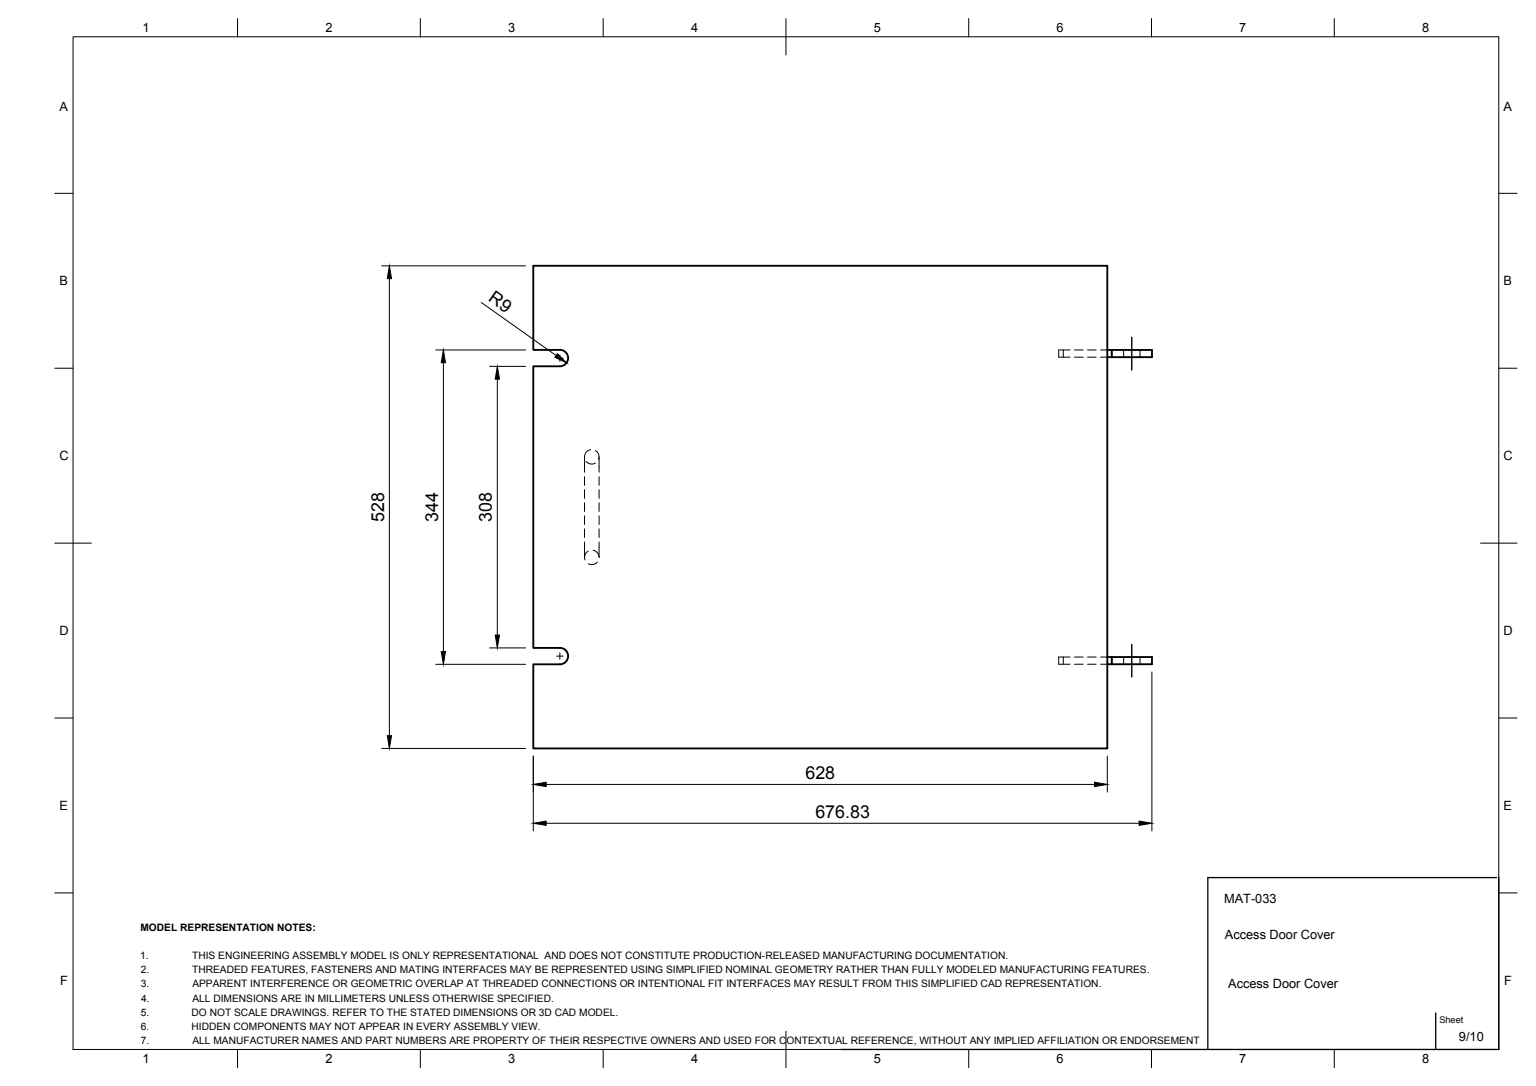
ISO-10303-21;
HEADER;
/* Generated by software containing ST-Developer
 * from STEP Tools, Inc. (www.steptools.com) 
 */

FILE_DESCRIPTION(
/* description */ ('STEP AP214'),
/* implementation_level */ '2;1');

FILE_NAME(
/* name */ 'Access Door Cover.step',
/* time_stamp */ '2026-11-14T07:13:32-08:00',
/* author */ (''),
/* organization */ (''),
/* preprocessor_version */ 'ST-DEVELOPER v20.2',
/* originating_system */ 'Autodesk Translation Framework v15.17.0.0',
/* authorisation */ '');

FILE_SCHEMA (('AUTOMOTIVE_DESIGN { 1 0 10303 214 3 1 1 }'));
ENDSEC;

DATA;
#10=MECHANICAL_DESIGN_GEOMETRIC_PRESENTATION_REPRESENTATION('',(#1315,#1316,#1317,#1318),#32903);
#639=TOROIDAL_SURFACE('',#16259,11.,7.93749999999998);
#640=TOROIDAL_SURFACE('',#16264,11.,7.93749999999998);
#675=SHAPE_REPRESENTATION_RELATIONSHIP('SRR','None',#33017,#689);
#689=ADVANCED_BREP_SHAPE_REPRESENTATION('',(#1404,#1405,#1406,#1407),#32892);
#856=CIRCLE('',#16214,9.00000000000001);
#857=CIRCLE('',#16215,9.00000000000001);
#858=CIRCLE('',#16220,9.00000000000001);
#859=CIRCLE('',#16221,9.00000000000001);
#860=CIRCLE('',#16230,9.00000000000001);
#861=CIRCLE('',#16231,9.00000000000001);
#862=CIRCLE('',#16233,5.);
#863=CIRCLE('',#16234,5.);
#864=CIRCLE('',#16236,22.);
#865=CIRCLE('',#16237,22.);
#866=CIRCLE('',#16245,9.00000000000001);
#867=CIRCLE('',#16246,9.00000000000001);
#868=CIRCLE('',#16248,5.);
#869=CIRCLE('',#16249,5.);
#870=CIRCLE('',#16251,22.);
#871=CIRCLE('',#16252,22.);
#872=CIRCLE('',#16260,7.93749999999998);
#873=CIRCLE('',#16261,3.06250000000001);
#874=CIRCLE('',#16262,7.93749999999998);
#875=CIRCLE('',#16263,7.93749999999998);
#876=CIRCLE('',#16265,7.93749999999998);
#877=CIRCLE('',#16266,3.06250000000001);
#878=CIRCLE('',#16267,7.93749999999998);
#879=CIRCLE('',#16268,7.93749999999998);
#880=CIRCLE('',#16270,7.93749999999998);
#881=CIRCLE('',#16273,7.93749999999998);
#1171=CYLINDRICAL_SURFACE('',#16213,9.00000000000001);
#1172=CYLINDRICAL_SURFACE('',#16219,9.00000000000001);
#1173=CYLINDRICAL_SURFACE('',#16229,9.00000000000001);
#1174=CYLINDRICAL_SURFACE('',#16232,5.);
#1175=CYLINDRICAL_SURFACE('',#16235,22.);
#1176=CYLINDRICAL_SURFACE('',#16244,9.00000000000001);
#1177=CYLINDRICAL_SURFACE('',#16247,5.);
#1178=CYLINDRICAL_SURFACE('',#16250,22.);
#1179=CYLINDRICAL_SURFACE('',#16269,7.93749999999998);
#1180=CYLINDRICAL_SURFACE('',#16271,7.93749999999999);
#1181=CYLINDRICAL_SURFACE('',#16272,7.93749999999998);
#1315=STYLED_ITEM('',(#33098),#1404);
#1316=STYLED_ITEM('',(#33098),#1405);
#1317=STYLED_ITEM('',(#33098),#1406);
#1318=STYLED_ITEM('',(#33098),#1407);
#1404=MANIFOLD_SOLID_BREP('Body1',#15563);
#1405=MANIFOLD_SOLID_BREP('Body2',#15564);
#1406=MANIFOLD_SOLID_BREP('Body3',#15565);
#1407=MANIFOLD_SOLID_BREP('Body4',#15566);
#1591=FACE_BOUND('',#2953,.T.);
#1592=FACE_BOUND('',#2955,.T.);
#1593=FACE_BOUND('',#2964,.T.);
#1594=FACE_BOUND('',#2966,.T.);
#1918=FACE_OUTER_BOUND('',#2935,.T.);
#1919=FACE_OUTER_BOUND('',#2936,.T.);
#1920=FACE_OUTER_BOUND('',#2937,.T.);
#1921=FACE_OUTER_BOUND('',#2938,.T.);
#1922=FACE_OUTER_BOUND('',#2939,.T.);
#1923=FACE_OUTER_BOUND('',#2940,.T.);
#1924=FACE_OUTER_BOUND('',#2941,.T.);
#1925=FACE_OUTER_BOUND('',#2942,.T.);
#1926=FACE_OUTER_BOUND('',#2943,.T.);
#1927=FACE_OUTER_BOUND('',#2944,.T.);
#1928=FACE_OUTER_BOUND('',#2945,.T.);
#1929=FACE_OUTER_BOUND('',#2946,.T.);
#1930=FACE_OUTER_BOUND('',#2947,.T.);
#1931=FACE_OUTER_BOUND('',#2948,.T.);
#1932=FACE_OUTER_BOUND('',#2949,.T.);
#1933=FACE_OUTER_BOUND('',#2950,.T.);
#1934=FACE_OUTER_BOUND('',#2951,.T.);
#1935=FACE_OUTER_BOUND('',#2952,.T.);
#1936=FACE_OUTER_BOUND('',#2954,.T.);
#1937=FACE_OUTER_BOUND('',#2956,.T.);
#1938=FACE_OUTER_BOUND('',#2957,.T.);
#1939=FACE_OUTER_BOUND('',#2958,.T.);
#1940=FACE_OUTER_BOUND('',#2959,.T.);
#1941=FACE_OUTER_BOUND('',#2960,.T.);
#1942=FACE_OUTER_BOUND('',#2961,.T.);
#1943=FACE_OUTER_BOUND('',#2962,.T.);
#1944=FACE_OUTER_BOUND('',#2963,.T.);
#1945=FACE_OUTER_BOUND('',#2965,.T.);
#1946=FACE_OUTER_BOUND('',#2967,.T.);
#1947=FACE_OUTER_BOUND('',#2968,.T.);
#1948=FACE_OUTER_BOUND('',#2969,.T.);
#1949=FACE_OUTER_BOUND('',#2970,.T.);
#1950=FACE_OUTER_BOUND('',#2971,.T.);
#1951=FACE_OUTER_BOUND('',#2972,.T.);
#1952=FACE_OUTER_BOUND('',#2973,.T.);
#1953=FACE_OUTER_BOUND('',#2974,.T.);
#1954=FACE_OUTER_BOUND('',#2975,.T.);
#1955=FACE_OUTER_BOUND('',#2976,.T.);
#1956=FACE_OUTER_BOUND('',#2977,.T.);
#2935=EDGE_LOOP('',(#11071,#11072,#11073,#11074));
#2936=EDGE_LOOP('',(#11075,#11076,#11077,#11078));
#2937=EDGE_LOOP('',(#11079,#11080,#11081,#11082));
#2938=EDGE_LOOP('',(#11083,#11084,#11085,#11086));
#2939=EDGE_LOOP('',(#11087,#11088,#11089,#11090));
#2940=EDGE_LOOP('',(#11091,#11092,#11093,#11094));
#2941=EDGE_LOOP('',(#11095,#11096,#11097,#11098));
#2942=EDGE_LOOP('',(#11099,#11100,#11101,#11102));
#2943=EDGE_LOOP('',(#11103,#11104,#11105,#11106));
#2944=EDGE_LOOP('',(#11107,#11108,#11109,#11110));
#2945=EDGE_LOOP('',(#11111,#11112,#11113,#11114));
#2946=EDGE_LOOP('',(#11115,#11116,#11117,#11118));
#2947=EDGE_LOOP('',(#11119,#11120,#11121,#11122,#11123,#11124,#11125,#11126,
#11127,#11128,#11129,#11130));
#2948=EDGE_LOOP('',(#11131,#11132,#11133,#11134,#11135,#11136,#11137,#11138,
#11139,#11140,#11141,#11142));
#2949=EDGE_LOOP('',(#11143,#11144,#11145,#11146));
#2950=EDGE_LOOP('',(#11147,#11148,#11149,#11150));
#2951=EDGE_LOOP('',(#11151,#11152,#11153,#11154));
#2952=EDGE_LOOP('',(#11155,#11156,#11157,#11158,#11159,#11160));
#2953=EDGE_LOOP('',(#11161));
#2954=EDGE_LOOP('',(#11162,#11163,#11164,#11165,#11166,#11167));
#2955=EDGE_LOOP('',(#11168));
#2956=EDGE_LOOP('',(#11169,#11170,#11171,#11172));
#2957=EDGE_LOOP('',(#11173,#11174,#11175,#11176));
#2958=EDGE_LOOP('',(#11177,#11178,#11179,#11180));
#2959=EDGE_LOOP('',(#11181,#11182,#11183,#11184));
#2960=EDGE_LOOP('',(#11185,#11186,#11187,#11188));
#2961=EDGE_LOOP('',(#11189,#11190,#11191,#11192));
#2962=EDGE_LOOP('',(#11193,#11194,#11195,#11196));
#2963=EDGE_LOOP('',(#11197,#11198,#11199,#11200,#11201,#11202));
#2964=EDGE_LOOP('',(#11203));
#2965=EDGE_LOOP('',(#11204,#11205,#11206,#11207,#11208,#11209));
#2966=EDGE_LOOP('',(#11210));
#2967=EDGE_LOOP('',(#11211,#11212,#11213,#11214));
#2968=EDGE_LOOP('',(#11215,#11216,#11217,#11218));
#2969=EDGE_LOOP('',(#11219,#11220,#11221,#11222));
#2970=EDGE_LOOP('',(#11223,#11224,#11225,#11226));
#2971=EDGE_LOOP('',(#11227,#11228,#11229,#11230,#11231));
#2972=EDGE_LOOP('',(#11232,#11233,#11234,#11235,#11236));
#2973=EDGE_LOOP('',(#11237,#11238,#11239,#11240));
#2974=EDGE_LOOP('',(#11241,#11242,#11243,#11244,#11245,#11246));
#2975=EDGE_LOOP('',(#11247,#11248,#11249,#11250));
#2976=EDGE_LOOP('',(#11251));
#2977=EDGE_LOOP('',(#11252));
#4075=LINE('',#22530,#5479);
#4076=LINE('',#22532,#5480);
#4077=LINE('',#22534,#5481);
#4078=LINE('',#22535,#5482);
#4079=LINE('',#22538,#5483);
#4080=LINE('',#22540,#5484);
#4081=LINE('',#22541,#5485);
#4082=LINE('',#22546,#5486);
#4083=LINE('',#22550,#5487);
#4084=LINE('',#22552,#5488);
#4085=LINE('',#22553,#5489);
#4086=LINE('',#22556,#5490);
#4087=LINE('',#22558,#5491);
#4088=LINE('',#22559,#5492);
#4089=LINE('',#22562,#5493);
#4090=LINE('',#22564,#5494);
#4091=LINE('',#22565,#5495);
#4092=LINE('',#22570,#5496);
#4093=LINE('',#22574,#5497);
#4094=LINE('',#22576,#5498);
#4095=LINE('',#22577,#5499);
#4096=LINE('',#22580,#5500);
#4097=LINE('',#22582,#5501);
#4098=LINE('',#22583,#5502);
#4099=LINE('',#22586,#5503);
#4100=LINE('',#22588,#5504);
#4101=LINE('',#22589,#5505);
#4102=LINE('',#22592,#5506);
#4103=LINE('',#22594,#5507);
#4104=LINE('',#22595,#5508);
#4105=LINE('',#22597,#5509);
#4106=LINE('',#22598,#5510);
#4107=LINE('',#22605,#5511);
#4108=LINE('',#22612,#5512);
#4109=LINE('',#22615,#5513);
#4110=LINE('',#22620,#5514);
#4111=LINE('',#22624,#5515);
#4112=LINE('',#22626,#5516);
#4113=LINE('',#22628,#5517);
#4114=LINE('',#22629,#5518);
#4115=LINE('',#22632,#5519);
#4116=LINE('',#22634,#5520);
#4117=LINE('',#22636,#5521);
#4118=LINE('',#22637,#5522);
#4119=LINE('',#22639,#5523);
#4120=LINE('',#22641,#5524);
#4121=LINE('',#22643,#5525);
#4122=LINE('',#22649,#5526);
#4123=LINE('',#22656,#5527);
#4124=LINE('',#22659,#5528);
#4125=LINE('',#22665,#5529);
#4126=LINE('',#22668,#5530);
#4127=LINE('',#22670,#5531);
#4128=LINE('',#22672,#5532);
#4129=LINE('',#22673,#5533);
#4130=LINE('',#22676,#5534);
#4131=LINE('',#22678,#5535);
#4132=LINE('',#22680,#5536);
#4133=LINE('',#22681,#5537);
#4134=LINE('',#22683,#5538);
#4135=LINE('',#22685,#5539);
#4136=LINE('',#22687,#5540);
#4137=LINE('',#22707,#5541);
#4138=LINE('',#22710,#5542);
#4139=LINE('',#22714,#5543);
#5479=VECTOR('',#18417,1000.);
#5480=VECTOR('',#18418,1000.);
#5481=VECTOR('',#18419,1000.);
#5482=VECTOR('',#18420,1000.);
#5483=VECTOR('',#18423,1000.);
#5484=VECTOR('',#18424,1000.);
#5485=VECTOR('',#18425,1000.);
#5486=VECTOR('',#18430,1000.);
#5487=VECTOR('',#18435,1000.);
#5488=VECTOR('',#18436,1000.);
#5489=VECTOR('',#18437,1000.);
#5490=VECTOR('',#18440,1000.);
#5491=VECTOR('',#18441,1000.);
#5492=VECTOR('',#18442,1000.);
#5493=VECTOR('',#18445,1000.);
#5494=VECTOR('',#18446,1000.);
#5495=VECTOR('',#18447,1000.);
#5496=VECTOR('',#18452,1000.);
#5497=VECTOR('',#18457,1000.);
#5498=VECTOR('',#18458,1000.);
#5499=VECTOR('',#18459,1000.);
#5500=VECTOR('',#18462,1000.);
#5501=VECTOR('',#18463,1000.);
#5502=VECTOR('',#18464,1000.);
#5503=VECTOR('',#18467,1000.);
#5504=VECTOR('',#18468,1000.);
#5505=VECTOR('',#18469,1000.);
#5506=VECTOR('',#18472,1000.);
#5507=VECTOR('',#18473,1000.);
#5508=VECTOR('',#18474,1000.);
#5509=VECTOR('',#18477,1000.);
#5510=VECTOR('',#18478,1000.);
#5511=VECTOR('',#18487,9.00000000000001);
#5512=VECTOR('',#18494,1000.);
#5513=VECTOR('',#18497,1000.);
#5514=VECTOR('',#18502,1000.);
#5515=VECTOR('',#18507,1000.);
#5516=VECTOR('',#18508,1000.);
#5517=VECTOR('',#18509,1000.);
#5518=VECTOR('',#18510,1000.);
#5519=VECTOR('',#18513,1000.);
#5520=VECTOR('',#18514,1000.);
#5521=VECTOR('',#18515,1000.);
#5522=VECTOR('',#18516,1000.);
#5523=VECTOR('',#18519,1000.);
#5524=VECTOR('',#18522,1000.);
#5525=VECTOR('',#18525,1000.);
#5526=VECTOR('',#18532,9.00000000000001);
#5527=VECTOR('',#18539,1000.);
#5528=VECTOR('',#18542,1000.);
#5529=VECTOR('',#18549,1000.);
#5530=VECTOR('',#18552,1000.);
#5531=VECTOR('',#18553,1000.);
#5532=VECTOR('',#18554,1000.);
#5533=VECTOR('',#18555,1000.);
#5534=VECTOR('',#18558,1000.);
#5535=VECTOR('',#18559,1000.);
#5536=VECTOR('',#18560,1000.);
#5537=VECTOR('',#18561,1000.);
#5538=VECTOR('',#18564,1000.);
#5539=VECTOR('',#18567,1000.);
#5540=VECTOR('',#18570,1000.);
#5541=VECTOR('',#18595,7.93749999999998);
#5542=VECTOR('',#18600,7.93749999999999);
#5543=VECTOR('',#18605,7.93749999999998);
#6869=VERTEX_POINT('',#22528);
#6870=VERTEX_POINT('',#22529);
#6871=VERTEX_POINT('',#22531);
#6872=VERTEX_POINT('',#22533);
#6873=VERTEX_POINT('',#22537);
#6874=VERTEX_POINT('',#22539);
#6875=VERTEX_POINT('',#22543);
#6876=VERTEX_POINT('',#22545);
#6877=VERTEX_POINT('',#22549);
#6878=VERTEX_POINT('',#22551);
#6879=VERTEX_POINT('',#22555);
#6880=VERTEX_POINT('',#22557);
#6881=VERTEX_POINT('',#22561);
#6882=VERTEX_POINT('',#22563);
#6883=VERTEX_POINT('',#22567);
#6884=VERTEX_POINT('',#22569);
#6885=VERTEX_POINT('',#22573);
#6886=VERTEX_POINT('',#22575);
#6887=VERTEX_POINT('',#22579);
#6888=VERTEX_POINT('',#22581);
#6889=VERTEX_POINT('',#22585);
#6890=VERTEX_POINT('',#22587);
#6891=VERTEX_POINT('',#22591);
#6892=VERTEX_POINT('',#22593);
#6893=VERTEX_POINT('',#22602);
#6894=VERTEX_POINT('',#22604);
#6895=VERTEX_POINT('',#22608);
#6896=VERTEX_POINT('',#22609);
#6897=VERTEX_POINT('',#22611);
#6898=VERTEX_POINT('',#22613);
#6899=VERTEX_POINT('',#22617);
#6900=VERTEX_POINT('',#22619);
#6901=VERTEX_POINT('',#22623);
#6902=VERTEX_POINT('',#22625);
#6903=VERTEX_POINT('',#22627);
#6904=VERTEX_POINT('',#22631);
#6905=VERTEX_POINT('',#22633);
#6906=VERTEX_POINT('',#22635);
#6907=VERTEX_POINT('',#22646);
#6908=VERTEX_POINT('',#22648);
#6909=VERTEX_POINT('',#22652);
#6910=VERTEX_POINT('',#22653);
#6911=VERTEX_POINT('',#22655);
#6912=VERTEX_POINT('',#22657);
#6913=VERTEX_POINT('',#22661);
#6914=VERTEX_POINT('',#22663);
#6915=VERTEX_POINT('',#22667);
#6916=VERTEX_POINT('',#22669);
#6917=VERTEX_POINT('',#22671);
#6918=VERTEX_POINT('',#22675);
#6919=VERTEX_POINT('',#22677);
#6920=VERTEX_POINT('',#22679);
#6921=VERTEX_POINT('',#22690);
#6922=VERTEX_POINT('',#22691);
#6923=VERTEX_POINT('',#22693);
#6924=VERTEX_POINT('',#22698);
#6925=VERTEX_POINT('',#22700);
#6926=VERTEX_POINT('',#22702);
#6927=VERTEX_POINT('',#22706);
#6928=VERTEX_POINT('',#22712);
#8419=EDGE_CURVE('',#6869,#6870,#4075,.T.);
#8420=EDGE_CURVE('',#6871,#6869,#4076,.T.);
#8421=EDGE_CURVE('',#6871,#6872,#4077,.T.);
#8422=EDGE_CURVE('',#6872,#6870,#4078,.T.);
#8423=EDGE_CURVE('',#6873,#6869,#4079,.T.);
#8424=EDGE_CURVE('',#6874,#6873,#4080,.T.);
#8425=EDGE_CURVE('',#6874,#6871,#4081,.T.);
#8426=EDGE_CURVE('',#6875,#6873,#856,.T.);
#8427=EDGE_CURVE('',#6876,#6875,#4082,.T.);
#8428=EDGE_CURVE('',#6876,#6874,#857,.T.);
#8429=EDGE_CURVE('',#6877,#6875,#4083,.T.);
#8430=EDGE_CURVE('',#6878,#6877,#4084,.T.);
#8431=EDGE_CURVE('',#6878,#6876,#4085,.T.);
#8432=EDGE_CURVE('',#6879,#6877,#4086,.T.);
#8433=EDGE_CURVE('',#6880,#6879,#4087,.T.);
#8434=EDGE_CURVE('',#6880,#6878,#4088,.T.);
#8435=EDGE_CURVE('',#6881,#6879,#4089,.T.);
#8436=EDGE_CURVE('',#6882,#6881,#4090,.T.);
#8437=EDGE_CURVE('',#6882,#6880,#4091,.T.);
#8438=EDGE_CURVE('',#6883,#6881,#858,.T.);
#8439=EDGE_CURVE('',#6884,#6883,#4092,.T.);
#8440=EDGE_CURVE('',#6884,#6882,#859,.T.);
#8441=EDGE_CURVE('',#6885,#6883,#4093,.T.);
#8442=EDGE_CURVE('',#6886,#6885,#4094,.T.);
#8443=EDGE_CURVE('',#6886,#6884,#4095,.T.);
#8444=EDGE_CURVE('',#6887,#6885,#4096,.T.);
#8445=EDGE_CURVE('',#6888,#6887,#4097,.T.);
#8446=EDGE_CURVE('',#6888,#6886,#4098,.T.);
#8447=EDGE_CURVE('',#6889,#6887,#4099,.T.);
#8448=EDGE_CURVE('',#6890,#6889,#4100,.T.);
#8449=EDGE_CURVE('',#6890,#6888,#4101,.T.);
#8450=EDGE_CURVE('',#6891,#6889,#4102,.T.);
#8451=EDGE_CURVE('',#6892,#6891,#4103,.T.);
#8452=EDGE_CURVE('',#6892,#6890,#4104,.T.);
#8453=EDGE_CURVE('',#6870,#6891,#4105,.T.);
#8454=EDGE_CURVE('',#6872,#6892,#4106,.T.);
#8455=EDGE_CURVE('',#6893,#6893,#860,.T.);
#8456=EDGE_CURVE('',#6893,#6894,#4107,.T.);
#8457=EDGE_CURVE('',#6894,#6894,#861,.T.);
#8458=EDGE_CURVE('',#6895,#6896,#862,.T.);
#8459=EDGE_CURVE('',#6895,#6897,#4108,.T.);
#8460=EDGE_CURVE('',#6897,#6898,#863,.T.);
#8461=EDGE_CURVE('',#6896,#6898,#4109,.T.);
#8462=EDGE_CURVE('',#6899,#6895,#864,.T.);
#8463=EDGE_CURVE('',#6899,#6900,#4110,.T.);
#8464=EDGE_CURVE('',#6900,#6897,#865,.T.);
#8465=EDGE_CURVE('',#6896,#6901,#4111,.T.);
#8466=EDGE_CURVE('',#6901,#6902,#4112,.T.);
#8467=EDGE_CURVE('',#6902,#6903,#4113,.T.);
#8468=EDGE_CURVE('',#6903,#6899,#4114,.T.);
#8469=EDGE_CURVE('',#6904,#6900,#4115,.T.);
#8470=EDGE_CURVE('',#6905,#6904,#4116,.T.);
#8471=EDGE_CURVE('',#6906,#6905,#4117,.T.);
#8472=EDGE_CURVE('',#6898,#6906,#4118,.T.);
#8473=EDGE_CURVE('',#6901,#6906,#4119,.T.);
#8474=EDGE_CURVE('',#6902,#6905,#4120,.T.);
#8475=EDGE_CURVE('',#6903,#6904,#4121,.T.);
#8476=EDGE_CURVE('',#6907,#6907,#866,.T.);
#8477=EDGE_CURVE('',#6907,#6908,#4122,.T.);
#8478=EDGE_CURVE('',#6908,#6908,#867,.T.);
#8479=EDGE_CURVE('',#6909,#6910,#868,.T.);
#8480=EDGE_CURVE('',#6910,#6911,#4123,.T.);
#8481=EDGE_CURVE('',#6912,#6911,#869,.T.);
#8482=EDGE_CURVE('',#6909,#6912,#4124,.T.);
#8483=EDGE_CURVE('',#6913,#6909,#870,.T.);
#8484=EDGE_CURVE('',#6914,#6912,#871,.T.);
#8485=EDGE_CURVE('',#6913,#6914,#4125,.T.);
#8486=EDGE_CURVE('',#6915,#6913,#4126,.T.);
#8487=EDGE_CURVE('',#6916,#6915,#4127,.T.);
#8488=EDGE_CURVE('',#6917,#6916,#4128,.T.);
#8489=EDGE_CURVE('',#6910,#6917,#4129,.T.);
#8490=EDGE_CURVE('',#6911,#6918,#4130,.T.);
#8491=EDGE_CURVE('',#6918,#6919,#4131,.T.);
#8492=EDGE_CURVE('',#6919,#6920,#4132,.T.);
#8493=EDGE_CURVE('',#6920,#6914,#4133,.T.);
#8494=EDGE_CURVE('',#6917,#6918,#4134,.T.);
#8495=EDGE_CURVE('',#6916,#6919,#4135,.T.);
#8496=EDGE_CURVE('',#6915,#6920,#4136,.T.);
#8497=EDGE_CURVE('',#6921,#6922,#872,.T.);
#8498=EDGE_CURVE('',#6922,#6923,#873,.T.);
#8499=EDGE_CURVE('',#6923,#6923,#874,.T.);
#8500=EDGE_CURVE('',#6922,#6921,#875,.T.);
#8501=EDGE_CURVE('',#6924,#6924,#876,.T.);
#8502=EDGE_CURVE('',#6924,#6925,#877,.T.);
#8503=EDGE_CURVE('',#6926,#6925,#878,.T.);
#8504=EDGE_CURVE('',#6925,#6926,#879,.T.);
#8505=EDGE_CURVE('',#6923,#6927,#4137,.T.);
#8506=EDGE_CURVE('',#6927,#6927,#880,.T.);
#8507=EDGE_CURVE('',#6926,#6921,#4138,.T.);
#8508=EDGE_CURVE('',#6928,#6928,#881,.T.);
#8509=EDGE_CURVE('',#6928,#6924,#4139,.T.);
#11071=ORIENTED_EDGE('',*,*,#8419,.F.);
#11072=ORIENTED_EDGE('',*,*,#8420,.F.);
#11073=ORIENTED_EDGE('',*,*,#8421,.T.);
#11074=ORIENTED_EDGE('',*,*,#8422,.T.);
#11075=ORIENTED_EDGE('',*,*,#8423,.F.);
#11076=ORIENTED_EDGE('',*,*,#8424,.F.);
#11077=ORIENTED_EDGE('',*,*,#8425,.T.);
#11078=ORIENTED_EDGE('',*,*,#8420,.T.);
#11079=ORIENTED_EDGE('',*,*,#8426,.F.);
#11080=ORIENTED_EDGE('',*,*,#8427,.F.);
#11081=ORIENTED_EDGE('',*,*,#8428,.T.);
#11082=ORIENTED_EDGE('',*,*,#8424,.T.);
#11083=ORIENTED_EDGE('',*,*,#8429,.F.);
#11084=ORIENTED_EDGE('',*,*,#8430,.F.);
#11085=ORIENTED_EDGE('',*,*,#8431,.T.);
#11086=ORIENTED_EDGE('',*,*,#8427,.T.);
#11087=ORIENTED_EDGE('',*,*,#8432,.F.);
#11088=ORIENTED_EDGE('',*,*,#8433,.F.);
#11089=ORIENTED_EDGE('',*,*,#8434,.T.);
#11090=ORIENTED_EDGE('',*,*,#8430,.T.);
#11091=ORIENTED_EDGE('',*,*,#8435,.F.);
#11092=ORIENTED_EDGE('',*,*,#8436,.F.);
#11093=ORIENTED_EDGE('',*,*,#8437,.T.);
#11094=ORIENTED_EDGE('',*,*,#8433,.T.);
#11095=ORIENTED_EDGE('',*,*,#8438,.F.);
#11096=ORIENTED_EDGE('',*,*,#8439,.F.);
#11097=ORIENTED_EDGE('',*,*,#8440,.T.);
#11098=ORIENTED_EDGE('',*,*,#8436,.T.);
#11099=ORIENTED_EDGE('',*,*,#8441,.F.);
#11100=ORIENTED_EDGE('',*,*,#8442,.F.);
#11101=ORIENTED_EDGE('',*,*,#8443,.T.);
#11102=ORIENTED_EDGE('',*,*,#8439,.T.);
#11103=ORIENTED_EDGE('',*,*,#8444,.F.);
#11104=ORIENTED_EDGE('',*,*,#8445,.F.);
#11105=ORIENTED_EDGE('',*,*,#8446,.T.);
#11106=ORIENTED_EDGE('',*,*,#8442,.T.);
#11107=ORIENTED_EDGE('',*,*,#8447,.F.);
#11108=ORIENTED_EDGE('',*,*,#8448,.F.);
#11109=ORIENTED_EDGE('',*,*,#8449,.T.);
#11110=ORIENTED_EDGE('',*,*,#8445,.T.);
#11111=ORIENTED_EDGE('',*,*,#8450,.F.);
#11112=ORIENTED_EDGE('',*,*,#8451,.F.);
#11113=ORIENTED_EDGE('',*,*,#8452,.T.);
#11114=ORIENTED_EDGE('',*,*,#8448,.T.);
#11115=ORIENTED_EDGE('',*,*,#8453,.F.);
#11116=ORIENTED_EDGE('',*,*,#8422,.F.);
#11117=ORIENTED_EDGE('',*,*,#8454,.T.);
#11118=ORIENTED_EDGE('',*,*,#8451,.T.);
#11119=ORIENTED_EDGE('',*,*,#8421,.F.);
#11120=ORIENTED_EDGE('',*,*,#8425,.F.);
#11121=ORIENTED_EDGE('',*,*,#8428,.F.);
#11122=ORIENTED_EDGE('',*,*,#8431,.F.);
#11123=ORIENTED_EDGE('',*,*,#8434,.F.);
#11124=ORIENTED_EDGE('',*,*,#8437,.F.);
#11125=ORIENTED_EDGE('',*,*,#8440,.F.);
#11126=ORIENTED_EDGE('',*,*,#8443,.F.);
#11127=ORIENTED_EDGE('',*,*,#8446,.F.);
#11128=ORIENTED_EDGE('',*,*,#8449,.F.);
#11129=ORIENTED_EDGE('',*,*,#8452,.F.);
#11130=ORIENTED_EDGE('',*,*,#8454,.F.);
#11131=ORIENTED_EDGE('',*,*,#8419,.T.);
#11132=ORIENTED_EDGE('',*,*,#8453,.T.);
#11133=ORIENTED_EDGE('',*,*,#8450,.T.);
#11134=ORIENTED_EDGE('',*,*,#8447,.T.);
#11135=ORIENTED_EDGE('',*,*,#8444,.T.);
#11136=ORIENTED_EDGE('',*,*,#8441,.T.);
#11137=ORIENTED_EDGE('',*,*,#8438,.T.);
#11138=ORIENTED_EDGE('',*,*,#8435,.T.);
#11139=ORIENTED_EDGE('',*,*,#8432,.T.);
#11140=ORIENTED_EDGE('',*,*,#8429,.T.);
#11141=ORIENTED_EDGE('',*,*,#8426,.T.);
#11142=ORIENTED_EDGE('',*,*,#8423,.T.);
#11143=ORIENTED_EDGE('',*,*,#8455,.T.);
#11144=ORIENTED_EDGE('',*,*,#8456,.T.);
#11145=ORIENTED_EDGE('',*,*,#8457,.F.);
#11146=ORIENTED_EDGE('',*,*,#8456,.F.);
#11147=ORIENTED_EDGE('',*,*,#8458,.F.);
#11148=ORIENTED_EDGE('',*,*,#8459,.T.);
#11149=ORIENTED_EDGE('',*,*,#8460,.T.);
#11150=ORIENTED_EDGE('',*,*,#8461,.F.);
#11151=ORIENTED_EDGE('',*,*,#8462,.F.);
#11152=ORIENTED_EDGE('',*,*,#8463,.T.);
#11153=ORIENTED_EDGE('',*,*,#8464,.T.);
#11154=ORIENTED_EDGE('',*,*,#8459,.F.);
#11155=ORIENTED_EDGE('',*,*,#8462,.T.);
#11156=ORIENTED_EDGE('',*,*,#8458,.T.);
#11157=ORIENTED_EDGE('',*,*,#8465,.T.);
#11158=ORIENTED_EDGE('',*,*,#8466,.T.);
#11159=ORIENTED_EDGE('',*,*,#8467,.T.);
#11160=ORIENTED_EDGE('',*,*,#8468,.T.);
#11161=ORIENTED_EDGE('',*,*,#8455,.F.);
#11162=ORIENTED_EDGE('',*,*,#8464,.F.);
#11163=ORIENTED_EDGE('',*,*,#8469,.F.);
#11164=ORIENTED_EDGE('',*,*,#8470,.F.);
#11165=ORIENTED_EDGE('',*,*,#8471,.F.);
#11166=ORIENTED_EDGE('',*,*,#8472,.F.);
#11167=ORIENTED_EDGE('',*,*,#8460,.F.);
#11168=ORIENTED_EDGE('',*,*,#8457,.T.);
#11169=ORIENTED_EDGE('',*,*,#8472,.T.);
#11170=ORIENTED_EDGE('',*,*,#8473,.F.);
#11171=ORIENTED_EDGE('',*,*,#8465,.F.);
#11172=ORIENTED_EDGE('',*,*,#8461,.T.);
#11173=ORIENTED_EDGE('',*,*,#8471,.T.);
#11174=ORIENTED_EDGE('',*,*,#8474,.F.);
#11175=ORIENTED_EDGE('',*,*,#8466,.F.);
#11176=ORIENTED_EDGE('',*,*,#8473,.T.);
#11177=ORIENTED_EDGE('',*,*,#8470,.T.);
#11178=ORIENTED_EDGE('',*,*,#8475,.F.);
#11179=ORIENTED_EDGE('',*,*,#8467,.F.);
#11180=ORIENTED_EDGE('',*,*,#8474,.T.);
#11181=ORIENTED_EDGE('',*,*,#8469,.T.);
#11182=ORIENTED_EDGE('',*,*,#8463,.F.);
#11183=ORIENTED_EDGE('',*,*,#8468,.F.);
#11184=ORIENTED_EDGE('',*,*,#8475,.T.);
#11185=ORIENTED_EDGE('',*,*,#8476,.F.);
#11186=ORIENTED_EDGE('',*,*,#8477,.T.);
#11187=ORIENTED_EDGE('',*,*,#8478,.T.);
#11188=ORIENTED_EDGE('',*,*,#8477,.F.);
#11189=ORIENTED_EDGE('',*,*,#8479,.T.);
#11190=ORIENTED_EDGE('',*,*,#8480,.T.);
#11191=ORIENTED_EDGE('',*,*,#8481,.F.);
#11192=ORIENTED_EDGE('',*,*,#8482,.F.);
#11193=ORIENTED_EDGE('',*,*,#8483,.T.);
#11194=ORIENTED_EDGE('',*,*,#8482,.T.);
#11195=ORIENTED_EDGE('',*,*,#8484,.F.);
#11196=ORIENTED_EDGE('',*,*,#8485,.F.);
#11197=ORIENTED_EDGE('',*,*,#8483,.F.);
#11198=ORIENTED_EDGE('',*,*,#8486,.F.);
#11199=ORIENTED_EDGE('',*,*,#8487,.F.);
#11200=ORIENTED_EDGE('',*,*,#8488,.F.);
#11201=ORIENTED_EDGE('',*,*,#8489,.F.);
#11202=ORIENTED_EDGE('',*,*,#8479,.F.);
#11203=ORIENTED_EDGE('',*,*,#8476,.T.);
#11204=ORIENTED_EDGE('',*,*,#8484,.T.);
#11205=ORIENTED_EDGE('',*,*,#8481,.T.);
#11206=ORIENTED_EDGE('',*,*,#8490,.T.);
#11207=ORIENTED_EDGE('',*,*,#8491,.T.);
#11208=ORIENTED_EDGE('',*,*,#8492,.T.);
#11209=ORIENTED_EDGE('',*,*,#8493,.T.);
#11210=ORIENTED_EDGE('',*,*,#8478,.F.);
#11211=ORIENTED_EDGE('',*,*,#8490,.F.);
#11212=ORIENTED_EDGE('',*,*,#8480,.F.);
#11213=ORIENTED_EDGE('',*,*,#8489,.T.);
#11214=ORIENTED_EDGE('',*,*,#8494,.T.);
#11215=ORIENTED_EDGE('',*,*,#8491,.F.);
#11216=ORIENTED_EDGE('',*,*,#8494,.F.);
#11217=ORIENTED_EDGE('',*,*,#8488,.T.);
#11218=ORIENTED_EDGE('',*,*,#8495,.T.);
#11219=ORIENTED_EDGE('',*,*,#8492,.F.);
#11220=ORIENTED_EDGE('',*,*,#8495,.F.);
#11221=ORIENTED_EDGE('',*,*,#8487,.T.);
#11222=ORIENTED_EDGE('',*,*,#8496,.T.);
#11223=ORIENTED_EDGE('',*,*,#8493,.F.);
#11224=ORIENTED_EDGE('',*,*,#8496,.F.);
#11225=ORIENTED_EDGE('',*,*,#8486,.T.);
#11226=ORIENTED_EDGE('',*,*,#8485,.T.);
#11227=ORIENTED_EDGE('',*,*,#8497,.T.);
#11228=ORIENTED_EDGE('',*,*,#8498,.T.);
#11229=ORIENTED_EDGE('',*,*,#8499,.F.);
#11230=ORIENTED_EDGE('',*,*,#8498,.F.);
#11231=ORIENTED_EDGE('',*,*,#8500,.T.);
#11232=ORIENTED_EDGE('',*,*,#8501,.T.);
#11233=ORIENTED_EDGE('',*,*,#8502,.T.);
#11234=ORIENTED_EDGE('',*,*,#8503,.F.);
#11235=ORIENTED_EDGE('',*,*,#8504,.F.);
#11236=ORIENTED_EDGE('',*,*,#8502,.F.);
#11237=ORIENTED_EDGE('',*,*,#8499,.T.);
#11238=ORIENTED_EDGE('',*,*,#8505,.T.);
#11239=ORIENTED_EDGE('',*,*,#8506,.F.);
#11240=ORIENTED_EDGE('',*,*,#8505,.F.);
#11241=ORIENTED_EDGE('',*,*,#8503,.T.);
#11242=ORIENTED_EDGE('',*,*,#8504,.T.);
#11243=ORIENTED_EDGE('',*,*,#8507,.T.);
#11244=ORIENTED_EDGE('',*,*,#8500,.F.);
#11245=ORIENTED_EDGE('',*,*,#8497,.F.);
#11246=ORIENTED_EDGE('',*,*,#8507,.F.);
#11247=ORIENTED_EDGE('',*,*,#8508,.T.);
#11248=ORIENTED_EDGE('',*,*,#8509,.T.);
#11249=ORIENTED_EDGE('',*,*,#8501,.F.);
#11250=ORIENTED_EDGE('',*,*,#8509,.F.);
#11251=ORIENTED_EDGE('',*,*,#8508,.F.);
#11252=ORIENTED_EDGE('',*,*,#8506,.T.);
#14199=PLANE('',#16211);
#14200=PLANE('',#16212);
#14201=PLANE('',#16216);
#14202=PLANE('',#16217);
#14203=PLANE('',#16218);
#14204=PLANE('',#16222);
#14205=PLANE('',#16223);
#14206=PLANE('',#16224);
#14207=PLANE('',#16225);
#14208=PLANE('',#16226);
#14209=PLANE('',#16227);
#14210=PLANE('',#16228);
#14211=PLANE('',#16238);
#14212=PLANE('',#16239);
#14213=PLANE('',#16240);
#14214=PLANE('',#16241);
#14215=PLANE('',#16242);
#14216=PLANE('',#16243);
#14217=PLANE('',#16253);
#14218=PLANE('',#16254);
#14219=PLANE('',#16255);
#14220=PLANE('',#16256);
#14221=PLANE('',#16257);
#14222=PLANE('',#16258);
#14223=PLANE('',#16274);
#14224=PLANE('',#16275);
#14886=ADVANCED_FACE('',(#1918),#14199,.T.);
#14887=ADVANCED_FACE('',(#1919),#14200,.T.);
#14888=ADVANCED_FACE('',(#1920),#1171,.F.);
#14889=ADVANCED_FACE('',(#1921),#14201,.T.);
#14890=ADVANCED_FACE('',(#1922),#14202,.T.);
#14891=ADVANCED_FACE('',(#1923),#14203,.T.);
#14892=ADVANCED_FACE('',(#1924),#1172,.F.);
#14893=ADVANCED_FACE('',(#1925),#14204,.T.);
#14894=ADVANCED_FACE('',(#1926),#14205,.T.);
#14895=ADVANCED_FACE('',(#1927),#14206,.T.);
#14896=ADVANCED_FACE('',(#1928),#14207,.T.);
#14897=ADVANCED_FACE('',(#1929),#14208,.T.);
#14898=ADVANCED_FACE('',(#1930),#14209,.F.);
#14899=ADVANCED_FACE('',(#1931),#14210,.T.);
#14900=ADVANCED_FACE('',(#1932),#1173,.F.);
#14901=ADVANCED_FACE('',(#1933),#1174,.F.);
#14902=ADVANCED_FACE('',(#1934),#1175,.T.);
#14903=ADVANCED_FACE('',(#1935,#1591),#14211,.F.);
#14904=ADVANCED_FACE('',(#1936,#1592),#14212,.T.);
#14905=ADVANCED_FACE('',(#1937),#14213,.F.);
#14906=ADVANCED_FACE('',(#1938),#14214,.F.);
#14907=ADVANCED_FACE('',(#1939),#14215,.F.);
#14908=ADVANCED_FACE('',(#1940),#14216,.F.);
#14909=ADVANCED_FACE('',(#1941),#1176,.F.);
#14910=ADVANCED_FACE('',(#1942),#1177,.F.);
#14911=ADVANCED_FACE('',(#1943),#1178,.T.);
#14912=ADVANCED_FACE('',(#1944,#1593),#14217,.F.);
#14913=ADVANCED_FACE('',(#1945,#1594),#14218,.T.);
#14914=ADVANCED_FACE('',(#1946),#14219,.F.);
#14915=ADVANCED_FACE('',(#1947),#14220,.F.);
#14916=ADVANCED_FACE('',(#1948),#14221,.F.);
#14917=ADVANCED_FACE('',(#1949),#14222,.F.);
#14918=ADVANCED_FACE('',(#1950),#639,.T.);
#14919=ADVANCED_FACE('',(#1951),#640,.T.);
#14920=ADVANCED_FACE('',(#1952),#1179,.T.);
#14921=ADVANCED_FACE('',(#1953),#1180,.T.);
#14922=ADVANCED_FACE('',(#1954),#1181,.T.);
#14923=ADVANCED_FACE('',(#1955),#14223,.F.);
#14924=ADVANCED_FACE('',(#1956),#14224,.T.);
#15563=CLOSED_SHELL('',(#14886,#14887,#14888,#14889,#14890,#14891,#14892,
#14893,#14894,#14895,#14896,#14897,#14898,#14899));
#15564=CLOSED_SHELL('',(#14900,#14901,#14902,#14903,#14904,#14905,#14906,
#14907,#14908));
#15565=CLOSED_SHELL('',(#14909,#14910,#14911,#14912,#14913,#14914,#14915,
#14916,#14917));
#15566=CLOSED_SHELL('',(#14918,#14919,#14920,#14921,#14922,#14923,#14924));
#16210=AXIS2_PLACEMENT_3D('',#22526,#18413,#18414);
#16211=AXIS2_PLACEMENT_3D('',#22527,#18415,#18416);
#16212=AXIS2_PLACEMENT_3D('',#22536,#18421,#18422);
#16213=AXIS2_PLACEMENT_3D('',#22542,#18426,#18427);
#16214=AXIS2_PLACEMENT_3D('',#22544,#18428,#18429);
#16215=AXIS2_PLACEMENT_3D('',#22547,#18431,#18432);
#16216=AXIS2_PLACEMENT_3D('',#22548,#18433,#18434);
#16217=AXIS2_PLACEMENT_3D('',#22554,#18438,#18439);
#16218=AXIS2_PLACEMENT_3D('',#22560,#18443,#18444);
#16219=AXIS2_PLACEMENT_3D('',#22566,#18448,#18449);
#16220=AXIS2_PLACEMENT_3D('',#22568,#18450,#18451);
#16221=AXIS2_PLACEMENT_3D('',#22571,#18453,#18454);
#16222=AXIS2_PLACEMENT_3D('',#22572,#18455,#18456);
#16223=AXIS2_PLACEMENT_3D('',#22578,#18460,#18461);
#16224=AXIS2_PLACEMENT_3D('',#22584,#18465,#18466);
#16225=AXIS2_PLACEMENT_3D('',#22590,#18470,#18471);
#16226=AXIS2_PLACEMENT_3D('',#22596,#18475,#18476);
#16227=AXIS2_PLACEMENT_3D('',#22599,#18479,#18480);
#16228=AXIS2_PLACEMENT_3D('',#22600,#18481,#18482);
#16229=AXIS2_PLACEMENT_3D('',#22601,#18483,#18484);
#16230=AXIS2_PLACEMENT_3D('',#22603,#18485,#18486);
#16231=AXIS2_PLACEMENT_3D('',#22606,#18488,#18489);
#16232=AXIS2_PLACEMENT_3D('',#22607,#18490,#18491);
#16233=AXIS2_PLACEMENT_3D('',#22610,#18492,#18493);
#16234=AXIS2_PLACEMENT_3D('',#22614,#18495,#18496);
#16235=AXIS2_PLACEMENT_3D('',#22616,#18498,#18499);
#16236=AXIS2_PLACEMENT_3D('',#22618,#18500,#18501);
#16237=AXIS2_PLACEMENT_3D('',#22621,#18503,#18504);
#16238=AXIS2_PLACEMENT_3D('',#22622,#18505,#18506);
#16239=AXIS2_PLACEMENT_3D('',#22630,#18511,#18512);
#16240=AXIS2_PLACEMENT_3D('',#22638,#18517,#18518);
#16241=AXIS2_PLACEMENT_3D('',#22640,#18520,#18521);
#16242=AXIS2_PLACEMENT_3D('',#22642,#18523,#18524);
#16243=AXIS2_PLACEMENT_3D('',#22644,#18526,#18527);
#16244=AXIS2_PLACEMENT_3D('',#22645,#18528,#18529);
#16245=AXIS2_PLACEMENT_3D('',#22647,#18530,#18531);
#16246=AXIS2_PLACEMENT_3D('',#22650,#18533,#18534);
#16247=AXIS2_PLACEMENT_3D('',#22651,#18535,#18536);
#16248=AXIS2_PLACEMENT_3D('',#22654,#18537,#18538);
#16249=AXIS2_PLACEMENT_3D('',#22658,#18540,#18541);
#16250=AXIS2_PLACEMENT_3D('',#22660,#18543,#18544);
#16251=AXIS2_PLACEMENT_3D('',#22662,#18545,#18546);
#16252=AXIS2_PLACEMENT_3D('',#22664,#18547,#18548);
#16253=AXIS2_PLACEMENT_3D('',#22666,#18550,#18551);
#16254=AXIS2_PLACEMENT_3D('',#22674,#18556,#18557);
#16255=AXIS2_PLACEMENT_3D('',#22682,#18562,#18563);
#16256=AXIS2_PLACEMENT_3D('',#22684,#18565,#18566);
#16257=AXIS2_PLACEMENT_3D('',#22686,#18568,#18569);
#16258=AXIS2_PLACEMENT_3D('',#22688,#18571,#18572);
#16259=AXIS2_PLACEMENT_3D('',#22689,#18573,#18574);
#16260=AXIS2_PLACEMENT_3D('',#22692,#18575,#18576);
#16261=AXIS2_PLACEMENT_3D('',#22694,#18577,#18578);
#16262=AXIS2_PLACEMENT_3D('',#22695,#18579,#18580);
#16263=AXIS2_PLACEMENT_3D('',#22696,#18581,#18582);
#16264=AXIS2_PLACEMENT_3D('',#22697,#18583,#18584);
#16265=AXIS2_PLACEMENT_3D('',#22699,#18585,#18586);
#16266=AXIS2_PLACEMENT_3D('',#22701,#18587,#18588);
#16267=AXIS2_PLACEMENT_3D('',#22703,#18589,#18590);
#16268=AXIS2_PLACEMENT_3D('',#22704,#18591,#18592);
#16269=AXIS2_PLACEMENT_3D('',#22705,#18593,#18594);
#16270=AXIS2_PLACEMENT_3D('',#22708,#18596,#18597);
#16271=AXIS2_PLACEMENT_3D('',#22709,#18598,#18599);
#16272=AXIS2_PLACEMENT_3D('',#22711,#18601,#18602);
#16273=AXIS2_PLACEMENT_3D('',#22713,#18603,#18604);
#16274=AXIS2_PLACEMENT_3D('',#22715,#18606,#18607);
#16275=AXIS2_PLACEMENT_3D('',#22716,#18608,#18609);
#18413=DIRECTION('axis',(0.,0.,1.));
#18414=DIRECTION('refdir',(1.,0.,0.));
#18415=DIRECTION('center_axis',(1.,0.,-1.81014623580189E-15));
#18416=DIRECTION('ref_axis',(-1.81014623580189E-15,0.,-1.));
#18417=DIRECTION('',(-1.81014623580189E-15,0.,-1.));
#18418=DIRECTION('',(0.,1.,0.));
#18419=DIRECTION('',(-1.81014623580189E-15,0.,-1.));
#18420=DIRECTION('',(0.,1.,0.));
#18421=DIRECTION('center_axis',(0.,0.,1.));
#18422=DIRECTION('ref_axis',(1.,0.,0.));
#18423=DIRECTION('',(1.,0.,0.));
#18424=DIRECTION('',(0.,1.,0.));
#18425=DIRECTION('',(1.,0.,0.));
#18426=DIRECTION('center_axis',(0.,1.,0.));
#18427=DIRECTION('ref_axis',(0.,0.,1.));
#18428=DIRECTION('center_axis',(0.,-1.,0.));
#18429=DIRECTION('ref_axis',(0.,0.,1.));
#18430=DIRECTION('',(0.,1.,0.));
#18431=DIRECTION('center_axis',(0.,-1.,0.));
#18432=DIRECTION('ref_axis',(0.,0.,1.));
#18433=DIRECTION('center_axis',(-9.57088814332031E-16,0.,-1.));
#18434=DIRECTION('ref_axis',(-1.,0.,9.57088814332031E-16));
#18435=DIRECTION('',(-1.,0.,9.57088814332031E-16));
#18436=DIRECTION('',(0.,1.,0.));
#18437=DIRECTION('',(-1.,0.,9.57088814332031E-16));
#18438=DIRECTION('center_axis',(1.,0.,0.));
#18439=DIRECTION('ref_axis',(0.,0.,-1.));
#18440=DIRECTION('',(0.,0.,-1.));
#18441=DIRECTION('',(0.,1.,0.));
#18442=DIRECTION('',(0.,0.,-1.));
#18443=DIRECTION('center_axis',(0.,0.,1.));
#18444=DIRECTION('ref_axis',(1.,0.,0.));
#18445=DIRECTION('',(1.,0.,0.));
#18446=DIRECTION('',(0.,1.,0.));
#18447=DIRECTION('',(1.,0.,0.));
#18448=DIRECTION('center_axis',(0.,1.,0.));
#18449=DIRECTION('ref_axis',(0.,0.,1.));
#18450=DIRECTION('center_axis',(0.,-1.,0.));
#18451=DIRECTION('ref_axis',(0.,0.,1.));
#18452=DIRECTION('',(0.,1.,0.));
#18453=DIRECTION('center_axis',(0.,-1.,0.));
#18454=DIRECTION('ref_axis',(0.,0.,1.));
#18455=DIRECTION('center_axis',(0.,0.,-1.));
#18456=DIRECTION('ref_axis',(-1.,0.,0.));
#18457=DIRECTION('',(-1.,0.,0.));
#18458=DIRECTION('',(0.,1.,0.));
#18459=DIRECTION('',(-1.,0.,0.));
#18460=DIRECTION('center_axis',(1.,0.,1.81014623580188E-15));
#18461=DIRECTION('ref_axis',(1.81014623580188E-15,0.,-1.));
#18462=DIRECTION('',(1.81014623580188E-15,0.,-1.));
#18463=DIRECTION('',(0.,1.,0.));
#18464=DIRECTION('',(1.81014623580188E-15,0.,-1.));
#18465=DIRECTION('center_axis',(0.,0.,1.));
#18466=DIRECTION('ref_axis',(1.,0.,0.));
#18467=DIRECTION('',(1.,0.,0.));
#18468=DIRECTION('',(0.,1.,0.));
#18469=DIRECTION('',(1.,0.,0.));
#18470=DIRECTION('center_axis',(-1.,0.,0.));
#18471=DIRECTION('ref_axis',(0.,0.,1.));
#18472=DIRECTION('',(0.,0.,1.));
#18473=DIRECTION('',(0.,1.,0.));
#18474=DIRECTION('',(0.,0.,1.));
#18475=DIRECTION('center_axis',(0.,0.,-1.));
#18476=DIRECTION('ref_axis',(-1.,0.,0.));
#18477=DIRECTION('',(-1.,0.,0.));
#18478=DIRECTION('',(-1.,0.,0.));
#18479=DIRECTION('center_axis',(0.,1.,0.));
#18480=DIRECTION('ref_axis',(0.,0.,1.));
#18481=DIRECTION('center_axis',(0.,1.,0.));
#18482=DIRECTION('ref_axis',(0.,0.,1.));
#18483=DIRECTION('center_axis',(0.,0.,-1.));
#18484=DIRECTION('ref_axis',(-1.,0.,0.));
#18485=DIRECTION('center_axis',(0.,0.,1.));
#18486=DIRECTION('ref_axis',(1.,0.,0.));
#18487=DIRECTION('',(0.,0.,-1.));
#18488=DIRECTION('center_axis',(0.,0.,1.));
#18489=DIRECTION('ref_axis',(1.,0.,0.));
#18490=DIRECTION('center_axis',(0.,0.,-1.));
#18491=DIRECTION('ref_axis',(-1.,0.,0.));
#18492=DIRECTION('center_axis',(0.,0.,-1.));
#18493=DIRECTION('ref_axis',(1.,0.,0.));
#18494=DIRECTION('',(0.,0.,-1.));
#18495=DIRECTION('center_axis',(0.,0.,-1.));
#18496=DIRECTION('ref_axis',(1.,0.,0.));
#18497=DIRECTION('',(0.,0.,-1.));
#18498=DIRECTION('center_axis',(0.,0.,-1.));
#18499=DIRECTION('ref_axis',(-0.666666666666667,-0.74535599249993,0.));
#18500=DIRECTION('center_axis',(0.,0.,1.));
#18501=DIRECTION('ref_axis',(-1.,0.,0.));
#18502=DIRECTION('',(0.,0.,-1.));
#18503=DIRECTION('center_axis',(0.,0.,1.));
#18504=DIRECTION('ref_axis',(-1.,0.,0.));
#18505=DIRECTION('center_axis',(0.,0.,-1.));
#18506=DIRECTION('ref_axis',(-1.,0.,0.));
#18507=DIRECTION('',(1.,0.,0.));
#18508=DIRECTION('',(0.707106781186552,0.707106781186543,0.));
#18509=DIRECTION('',(-6.16790569236198E-15,1.,0.));
#18510=DIRECTION('',(-1.,0.,0.));
#18511=DIRECTION('center_axis',(0.,0.,-1.));
#18512=DIRECTION('ref_axis',(-1.,0.,0.));
#18513=DIRECTION('',(-1.,0.,0.));
#18514=DIRECTION('',(-6.16790569236198E-15,1.,0.));
#18515=DIRECTION('',(0.707106781186552,0.707106781186543,0.));
#18516=DIRECTION('',(1.,0.,0.));
#18517=DIRECTION('center_axis',(0.,1.,0.));
#18518=DIRECTION('ref_axis',(0.,0.,1.));
#18519=DIRECTION('',(0.,0.,-1.));
#18520=DIRECTION('center_axis',(-0.707106781186543,0.707106781186552,0.));
#18521=DIRECTION('ref_axis',(-0.707106781186552,-0.707106781186543,0.));
#18522=DIRECTION('',(0.,0.,-1.));
#18523=DIRECTION('center_axis',(-1.,-6.16790569236198E-15,0.));
#18524=DIRECTION('ref_axis',(6.16790569236198E-15,-1.,0.));
#18525=DIRECTION('',(0.,0.,-1.));
#18526=DIRECTION('center_axis',(0.,-1.,0.));
#18527=DIRECTION('ref_axis',(0.,0.,-1.));
#18528=DIRECTION('center_axis',(0.,0.,1.));
#18529=DIRECTION('ref_axis',(-1.,0.,0.));
#18530=DIRECTION('center_axis',(0.,0.,1.));
#18531=DIRECTION('ref_axis',(1.,0.,0.));
#18532=DIRECTION('',(0.,0.,1.));
#18533=DIRECTION('center_axis',(0.,0.,1.));
#18534=DIRECTION('ref_axis',(1.,0.,0.));
#18535=DIRECTION('center_axis',(0.,0.,1.));
#18536=DIRECTION('ref_axis',(-1.,0.,0.));
#18537=DIRECTION('center_axis',(0.,0.,-1.));
#18538=DIRECTION('ref_axis',(1.,0.,0.));
#18539=DIRECTION('',(0.,0.,1.));
#18540=DIRECTION('center_axis',(0.,0.,-1.));
#18541=DIRECTION('ref_axis',(1.,0.,0.));
#18542=DIRECTION('',(0.,0.,1.));
#18543=DIRECTION('center_axis',(0.,0.,1.));
#18544=DIRECTION('ref_axis',(-0.666666666666667,-0.74535599249993,0.));
#18545=DIRECTION('center_axis',(0.,0.,1.));
#18546=DIRECTION('ref_axis',(-1.,0.,0.));
#18547=DIRECTION('center_axis',(0.,0.,1.));
#18548=DIRECTION('ref_axis',(-1.,0.,0.));
#18549=DIRECTION('',(0.,0.,1.));
#18550=DIRECTION('center_axis',(0.,0.,1.));
#18551=DIRECTION('ref_axis',(-1.,0.,0.));
#18552=DIRECTION('',(-1.,0.,0.));
#18553=DIRECTION('',(-6.16790569236198E-15,1.,0.));
#18554=DIRECTION('',(0.707106781186552,0.707106781186543,0.));
#18555=DIRECTION('',(1.,0.,0.));
#18556=DIRECTION('center_axis',(0.,0.,1.));
#18557=DIRECTION('ref_axis',(-1.,0.,0.));
#18558=DIRECTION('',(1.,0.,0.));
#18559=DIRECTION('',(0.707106781186552,0.707106781186543,0.));
#18560=DIRECTION('',(-6.16790569236198E-15,1.,0.));
#18561=DIRECTION('',(-1.,0.,0.));
#18562=DIRECTION('center_axis',(0.,1.,0.));
#18563=DIRECTION('ref_axis',(0.,0.,-1.));
#18564=DIRECTION('',(0.,0.,1.));
#18565=DIRECTION('center_axis',(-0.707106781186543,0.707106781186552,0.));
#18566=DIRECTION('ref_axis',(-0.707106781186552,-0.707106781186543,0.));
#18567=DIRECTION('',(0.,0.,1.));
#18568=DIRECTION('center_axis',(-1.,-6.16790569236198E-15,0.));
#18569=DIRECTION('ref_axis',(6.16790569236198E-15,-1.,0.));
#18570=DIRECTION('',(0.,0.,1.));
#18571=DIRECTION('center_axis',(0.,-1.,0.));
#18572=DIRECTION('ref_axis',(0.,0.,1.));
#18573=DIRECTION('center_axis',(-1.,0.,0.));
#18574=DIRECTION('ref_axis',(0.,0.,1.));
#18575=DIRECTION('center_axis',(0.,4.44089209850063E-16,1.));
#18576=DIRECTION('ref_axis',(0.,-1.,4.44089209850063E-16));
#18577=DIRECTION('center_axis',(1.,0.,0.));
#18578=DIRECTION('ref_axis',(0.,0.,1.));
#18579=DIRECTION('center_axis',(0.,-1.,-1.60812264967664E-16));
#18580=DIRECTION('ref_axis',(0.,1.60812264967664E-16,-1.));
#18581=DIRECTION('center_axis',(0.,4.44089209850063E-16,1.));
#18582=DIRECTION('ref_axis',(0.,-1.,4.44089209850063E-16));
#18583=DIRECTION('center_axis',(-1.,0.,0.));
#18584=DIRECTION('ref_axis',(0.,0.,1.));
#18585=DIRECTION('center_axis',(0.,1.,-3.82856869892695E-16));
#18586=DIRECTION('ref_axis',(0.,3.82856869892695E-16,1.));
#18587=DIRECTION('center_axis',(1.,0.,0.));
#18588=DIRECTION('ref_axis',(0.,0.,1.));
#18589=DIRECTION('center_axis',(0.,4.44089209850063E-16,1.));
#18590=DIRECTION('ref_axis',(0.,-1.,4.44089209850063E-16));
#18591=DIRECTION('center_axis',(0.,4.44089209850063E-16,1.));
#18592=DIRECTION('ref_axis',(0.,-1.,4.44089209850063E-16));
#18593=DIRECTION('center_axis',(0.,1.,1.41610079671576E-16));
#18594=DIRECTION('ref_axis',(0.,-1.41610079671576E-16,1.));
#18595=DIRECTION('',(0.,-1.,-1.41610079671576E-16));
#18596=DIRECTION('center_axis',(0.,-1.,-1.60812264967664E-16));
#18597=DIRECTION('ref_axis',(0.,1.60812264967664E-16,-1.));
#18598=DIRECTION('center_axis',(0.,0.,-1.));
#18599=DIRECTION('ref_axis',(-1.,0.,0.));
#18600=DIRECTION('',(0.,0.,1.));
#18601=DIRECTION('center_axis',(0.,-1.,0.));
#18602=DIRECTION('ref_axis',(0.,0.,-1.));
#18603=DIRECTION('center_axis',(0.,1.,-3.82856869892695E-16));
#18604=DIRECTION('ref_axis',(0.,3.82856869892695E-16,1.));
#18605=DIRECTION('',(0.,1.,0.));
#18606=DIRECTION('center_axis',(0.,1.,-3.82856869892695E-16));
#18607=DIRECTION('ref_axis',(0.,3.82856869892695E-16,1.));
#18608=DIRECTION('center_axis',(0.,-1.,-1.60812264967664E-16));
#18609=DIRECTION('ref_axis',(0.,1.60812264967664E-16,-1.));
#22526=CARTESIAN_POINT('',(0.,0.,0.));
#22527=CARTESIAN_POINT('Origin',(314.,-7.9375,-264.));
#22528=CARTESIAN_POINT('',(314.,0.,-172.));
#22529=CARTESIAN_POINT('',(314.,0.,-264.));
#22530=CARTESIAN_POINT('',(314.,0.,-264.));
#22531=CARTESIAN_POINT('',(314.,-7.9375,-172.));
#22532=CARTESIAN_POINT('',(314.,-7.9375,-172.));
#22533=CARTESIAN_POINT('',(314.,-7.9375,-264.));
#22534=CARTESIAN_POINT('',(314.,-7.9375,-264.));
#22535=CARTESIAN_POINT('',(314.,-7.9375,-264.));
#22536=CARTESIAN_POINT('Origin',(314.,-7.9375,-172.));
#22537=CARTESIAN_POINT('',(285.,0.,-172.));
#22538=CARTESIAN_POINT('',(314.,0.,-172.));
#22539=CARTESIAN_POINT('',(285.,-7.9375,-172.));
#22540=CARTESIAN_POINT('',(285.,-7.9375,-172.));
#22541=CARTESIAN_POINT('',(314.,-7.9375,-172.));
#22542=CARTESIAN_POINT('Origin',(285.,-7.9375,-163.));
#22543=CARTESIAN_POINT('',(285.,0.,-154.));
#22544=CARTESIAN_POINT('Origin',(285.,0.,-163.));
#22545=CARTESIAN_POINT('',(285.,-7.9375,-154.));
#22546=CARTESIAN_POINT('',(285.,-7.9375,-154.));
#22547=CARTESIAN_POINT('Origin',(285.,-7.9375,-163.));
#22548=CARTESIAN_POINT('Origin',(285.,-7.9375,-154.));
#22549=CARTESIAN_POINT('',(314.,0.,-154.));
#22550=CARTESIAN_POINT('',(285.,0.,-154.));
#22551=CARTESIAN_POINT('',(314.,-7.9375,-154.));
#22552=CARTESIAN_POINT('',(314.,-7.9375,-154.));
#22553=CARTESIAN_POINT('',(285.,-7.9375,-154.));
#22554=CARTESIAN_POINT('Origin',(314.,-7.9375,-154.));
#22555=CARTESIAN_POINT('',(314.,0.,154.));
#22556=CARTESIAN_POINT('',(314.,0.,-154.));
#22557=CARTESIAN_POINT('',(314.,-7.9375,154.));
#22558=CARTESIAN_POINT('',(314.,-7.9375,154.));
#22559=CARTESIAN_POINT('',(314.,-7.9375,-154.));
#22560=CARTESIAN_POINT('Origin',(314.,-7.9375,154.));
#22561=CARTESIAN_POINT('',(285.,0.,154.));
#22562=CARTESIAN_POINT('',(314.,0.,154.));
#22563=CARTESIAN_POINT('',(285.,-7.9375,154.));
#22564=CARTESIAN_POINT('',(285.,-7.9375,154.));
#22565=CARTESIAN_POINT('',(314.,-7.9375,154.));
#22566=CARTESIAN_POINT('Origin',(285.,-7.9375,163.));
#22567=CARTESIAN_POINT('',(285.,0.,172.));
#22568=CARTESIAN_POINT('Origin',(285.,0.,163.));
#22569=CARTESIAN_POINT('',(285.,-7.9375,172.));
#22570=CARTESIAN_POINT('',(285.,-7.9375,172.));
#22571=CARTESIAN_POINT('Origin',(285.,-7.9375,163.));
#22572=CARTESIAN_POINT('Origin',(285.,-7.9375,172.));
#22573=CARTESIAN_POINT('',(314.,0.,172.));
#22574=CARTESIAN_POINT('',(285.,0.,172.));
#22575=CARTESIAN_POINT('',(314.,-7.9375,172.));
#22576=CARTESIAN_POINT('',(314.,-7.9375,172.));
#22577=CARTESIAN_POINT('',(285.,-7.9375,172.));
#22578=CARTESIAN_POINT('Origin',(314.,-7.9375,172.));
#22579=CARTESIAN_POINT('',(314.,0.,264.));
#22580=CARTESIAN_POINT('',(314.,0.,172.));
#22581=CARTESIAN_POINT('',(314.,-7.9375,264.));
#22582=CARTESIAN_POINT('',(314.,-7.9375,264.));
#22583=CARTESIAN_POINT('',(314.,-7.9375,172.));
#22584=CARTESIAN_POINT('Origin',(-314.,-7.9375,264.));
#22585=CARTESIAN_POINT('',(-314.,0.,264.));
#22586=CARTESIAN_POINT('',(-314.,0.,264.));
#22587=CARTESIAN_POINT('',(-314.,-7.9375,264.));
#22588=CARTESIAN_POINT('',(-314.,-7.9375,264.));
#22589=CARTESIAN_POINT('',(-314.,-7.9375,264.));
#22590=CARTESIAN_POINT('Origin',(-314.,-7.9375,264.));
#22591=CARTESIAN_POINT('',(-314.,0.,-264.));
#22592=CARTESIAN_POINT('',(-314.,0.,264.));
#22593=CARTESIAN_POINT('',(-314.,-7.9375,-264.));
#22594=CARTESIAN_POINT('',(-314.,-7.9375,-264.));
#22595=CARTESIAN_POINT('',(-314.,-7.9375,264.));
#22596=CARTESIAN_POINT('Origin',(-314.,-7.9375,-264.));
#22597=CARTESIAN_POINT('',(-314.,0.,-264.));
#22598=CARTESIAN_POINT('',(-314.,-7.9375,-264.));
#22599=CARTESIAN_POINT('Origin',(285.,-7.9375,-163.));
#22600=CARTESIAN_POINT('Origin',(285.,0.,-163.));
#22601=CARTESIAN_POINT('Origin',(-340.832815729998,-8.,171.9375));
#22602=CARTESIAN_POINT('',(-331.832815729998,-8.,171.9375));
#22603=CARTESIAN_POINT('Origin',(-340.832815729998,-8.,171.9375));
#22604=CARTESIAN_POINT('',(-331.832815729998,-8.,164.));
#22605=CARTESIAN_POINT('',(-331.832815729998,-8.,171.9375));
#22606=CARTESIAN_POINT('Origin',(-340.832815729998,-8.,164.));
#22607=CARTESIAN_POINT('Origin',(-314.,-5.,171.9375));
#22608=CARTESIAN_POINT('',(-318.96903995,-5.55555555555555,171.9375));
#22609=CARTESIAN_POINT('',(-314.,0.,171.9375));
#22610=CARTESIAN_POINT('Origin',(-314.,-5.,171.9375));
#22611=CARTESIAN_POINT('',(-318.96903995,-5.55555555555555,164.));
#22612=CARTESIAN_POINT('',(-318.96903995,-5.55555555555555,171.9375));
#22613=CARTESIAN_POINT('',(-314.,0.,164.));
#22614=CARTESIAN_POINT('Origin',(-314.,-5.,164.));
#22615=CARTESIAN_POINT('',(-314.,0.,171.9375));
#22616=CARTESIAN_POINT('Origin',(-340.832815729998,-8.,171.9375));
#22617=CARTESIAN_POINT('',(-340.832815729998,14.,171.9375));
#22618=CARTESIAN_POINT('Origin',(-340.832815729998,-8.,171.9375));
#22619=CARTESIAN_POINT('',(-340.832815729998,14.,164.));
#22620=CARTESIAN_POINT('',(-340.832815729998,14.,171.9375));
#22621=CARTESIAN_POINT('Origin',(-340.832815729998,-8.,164.));
#22622=CARTESIAN_POINT('Origin',(-340.832815729998,-8.,171.9375));
#22623=CARTESIAN_POINT('',(-265.832815729998,0.,171.9375));
#22624=CARTESIAN_POINT('',(-265.832815729998,0.,171.9375));
#22625=CARTESIAN_POINT('',(-260.832815729998,5.,171.9375));
#22626=CARTESIAN_POINT('',(-260.832815729998,5.,171.9375));
#22627=CARTESIAN_POINT('',(-260.832815729998,14.,171.9375));
#22628=CARTESIAN_POINT('',(-260.832815729998,14.,171.9375));
#22629=CARTESIAN_POINT('',(-340.832815729998,14.,171.9375));
#22630=CARTESIAN_POINT('Origin',(-340.832815729998,-8.,164.));
#22631=CARTESIAN_POINT('',(-260.832815729998,14.,164.));
#22632=CARTESIAN_POINT('',(-340.832815729998,14.,164.));
#22633=CARTESIAN_POINT('',(-260.832815729998,5.,164.));
#22634=CARTESIAN_POINT('',(-260.832815729998,14.,164.));
#22635=CARTESIAN_POINT('',(-265.832815729998,0.,164.));
#22636=CARTESIAN_POINT('',(-260.832815729998,5.,164.));
#22637=CARTESIAN_POINT('',(-265.832815729998,0.,164.));
#22638=CARTESIAN_POINT('Origin',(-265.832815729998,0.,171.9375));
#22639=CARTESIAN_POINT('',(-265.832815729998,0.,171.9375));
#22640=CARTESIAN_POINT('Origin',(-260.832815729998,5.,171.9375));
#22641=CARTESIAN_POINT('',(-260.832815729998,5.,171.9375));
#22642=CARTESIAN_POINT('Origin',(-260.832815729998,14.,171.9375));
#22643=CARTESIAN_POINT('',(-260.832815729998,14.,171.9375));
#22644=CARTESIAN_POINT('Origin',(-340.832815729998,14.,171.9375));
#22645=CARTESIAN_POINT('Origin',(-340.832815729998,-8.,-171.9375));
#22646=CARTESIAN_POINT('',(-331.832815729998,-8.,-171.9375));
#22647=CARTESIAN_POINT('Origin',(-340.832815729998,-8.,-171.9375));
#22648=CARTESIAN_POINT('',(-331.832815729998,-8.,-164.));
#22649=CARTESIAN_POINT('',(-331.832815729998,-8.,-171.9375));
#22650=CARTESIAN_POINT('Origin',(-340.832815729998,-8.,-164.));
#22651=CARTESIAN_POINT('Origin',(-314.,-5.,-171.9375));
#22652=CARTESIAN_POINT('',(-318.96903995,-5.55555555555555,-171.9375));
#22653=CARTESIAN_POINT('',(-314.,0.,-171.9375));
#22654=CARTESIAN_POINT('Origin',(-314.,-5.,-171.9375));
#22655=CARTESIAN_POINT('',(-314.,0.,-164.));
#22656=CARTESIAN_POINT('',(-314.,0.,-171.9375));
#22657=CARTESIAN_POINT('',(-318.96903995,-5.55555555555555,-164.));
#22658=CARTESIAN_POINT('Origin',(-314.,-5.,-164.));
#22659=CARTESIAN_POINT('',(-318.96903995,-5.55555555555555,-171.9375));
#22660=CARTESIAN_POINT('Origin',(-340.832815729998,-8.,-171.9375));
#22661=CARTESIAN_POINT('',(-340.832815729998,14.,-171.9375));
#22662=CARTESIAN_POINT('Origin',(-340.832815729998,-8.,-171.9375));
#22663=CARTESIAN_POINT('',(-340.832815729998,14.,-164.));
#22664=CARTESIAN_POINT('Origin',(-340.832815729998,-8.,-164.));
#22665=CARTESIAN_POINT('',(-340.832815729998,14.,-171.9375));
#22666=CARTESIAN_POINT('Origin',(-340.832815729998,-8.,-171.9375));
#22667=CARTESIAN_POINT('',(-260.832815729998,14.,-171.9375));
#22668=CARTESIAN_POINT('',(-340.832815729998,14.,-171.9375));
#22669=CARTESIAN_POINT('',(-260.832815729998,5.,-171.9375));
#22670=CARTESIAN_POINT('',(-260.832815729998,14.,-171.9375));
#22671=CARTESIAN_POINT('',(-265.832815729998,0.,-171.9375));
#22672=CARTESIAN_POINT('',(-260.832815729998,5.,-171.9375));
#22673=CARTESIAN_POINT('',(-265.832815729998,0.,-171.9375));
#22674=CARTESIAN_POINT('Origin',(-340.832815729998,-8.,-164.));
#22675=CARTESIAN_POINT('',(-265.832815729998,0.,-164.));
#22676=CARTESIAN_POINT('',(-265.832815729998,0.,-164.));
#22677=CARTESIAN_POINT('',(-260.832815729998,5.,-164.));
#22678=CARTESIAN_POINT('',(-260.832815729998,5.,-164.));
#22679=CARTESIAN_POINT('',(-260.832815729998,14.,-164.));
#22680=CARTESIAN_POINT('',(-260.832815729998,14.,-164.));
#22681=CARTESIAN_POINT('',(-340.832815729998,14.,-164.));
#22682=CARTESIAN_POINT('Origin',(-265.832815729998,0.,-171.9375));
#22683=CARTESIAN_POINT('',(-265.832815729998,0.,-171.9375));
#22684=CARTESIAN_POINT('Origin',(-260.832815729998,5.,-171.9375));
#22685=CARTESIAN_POINT('',(-260.832815729998,5.,-171.9375));
#22686=CARTESIAN_POINT('Origin',(-260.832815729998,14.,-171.9375));
#22687=CARTESIAN_POINT('',(-260.832815729998,14.,-171.9375));
#22688=CARTESIAN_POINT('Origin',(-340.832815729998,14.,-171.9375));
#22689=CARTESIAN_POINT('Origin',(250.,49.,44.));
#22690=CARTESIAN_POINT('',(257.9375,60.,44.));
#22691=CARTESIAN_POINT('',(250.,52.0625,44.));
#22692=CARTESIAN_POINT('Origin',(250.,60.,44.));
#22693=CARTESIAN_POINT('',(250.,49.,47.0625));
#22694=CARTESIAN_POINT('Origin',(250.,49.,44.));
#22695=CARTESIAN_POINT('Origin',(250.,49.,55.));
#22696=CARTESIAN_POINT('Origin',(250.,60.,44.));
#22697=CARTESIAN_POINT('Origin',(250.,49.,-44.));
#22698=CARTESIAN_POINT('',(250.,49.,-47.0625));
#22699=CARTESIAN_POINT('Origin',(250.,49.,-55.));
#22700=CARTESIAN_POINT('',(250.,52.0625,-44.));
#22701=CARTESIAN_POINT('Origin',(250.,49.,-44.));
#22702=CARTESIAN_POINT('',(257.9375,60.,-44.));
#22703=CARTESIAN_POINT('Origin',(250.,60.,-44.));
#22704=CARTESIAN_POINT('Origin',(250.,60.,-44.));
#22705=CARTESIAN_POINT('Origin',(250.,0.,55.));
#22706=CARTESIAN_POINT('',(250.,9.71612661605436E-16,47.0625));
#22707=CARTESIAN_POINT('',(250.,1.12403000739313E-15,47.0625));
#22708=CARTESIAN_POINT('Origin',(250.,0.,55.));
#22709=CARTESIAN_POINT('Origin',(250.,60.,44.));
#22710=CARTESIAN_POINT('',(257.9375,60.,44.));
#22711=CARTESIAN_POINT('Origin',(250.,49.,-55.));
#22712=CARTESIAN_POINT('',(250.,0.,-47.0625));
#22713=CARTESIAN_POINT('Origin',(250.,0.,-55.));
#22714=CARTESIAN_POINT('',(250.,49.,-47.0625));
#22715=CARTESIAN_POINT('Origin',(250.,0.,-55.));
#22716=CARTESIAN_POINT('Origin',(250.,0.,55.));
#32875=UNCERTAINTY_MEASURE_WITH_UNIT(LENGTH_MEASURE(0.01),#32904,
'DISTANCE_ACCURACY_VALUE',
'Maximum model space distance between geometric entities at asserted c
onnectivities');
#32886=UNCERTAINTY_MEASURE_WITH_UNIT(LENGTH_MEASURE(0.01),#32904,
'DISTANCE_ACCURACY_VALUE',
'Maximum model space distance between geometric entities at asserted c
onnectivities');
#32892=(
GEOMETRIC_REPRESENTATION_CONTEXT(3)
GLOBAL_UNCERTAINTY_ASSIGNED_CONTEXT((#32875))
GLOBAL_UNIT_ASSIGNED_CONTEXT((#32904,#32906,#32907))
REPRESENTATION_CONTEXT('','3D')
);
#32903=(
GEOMETRIC_REPRESENTATION_CONTEXT(3)
GLOBAL_UNCERTAINTY_ASSIGNED_CONTEXT((#32886))
GLOBAL_UNIT_ASSIGNED_CONTEXT((#32904,#32906,#32907))
REPRESENTATION_CONTEXT('','3D')
);
#32904=(
LENGTH_UNIT()
NAMED_UNIT(*)
SI_UNIT(.MILLI.,.METRE.)
);
#32906=(
NAMED_UNIT(*)
PLANE_ANGLE_UNIT()
SI_UNIT($,.RADIAN.)
);
#32907=(
NAMED_UNIT(*)
SI_UNIT($,.STERADIAN.)
SOLID_ANGLE_UNIT()
);
#32913=SHAPE_DEFINITION_REPRESENTATION(#32929,#33017);
#32929=PRODUCT_DEFINITION_SHAPE('',$,#33034);
#33017=SHAPE_REPRESENTATION('',(#16210),#32892);
#33028=PRODUCT_DEFINITION_CONTEXT('part definition',#33078,'design');
#33034=PRODUCT_DEFINITION('Access Door Cover','Access Door Cover',#33050,
#33028);
#33050=PRODUCT_DEFINITION_FORMATION('',$,#33085);
#33078=APPLICATION_CONTEXT(
'Core Data for Automotive Mechanical Design Process');
#33079=PRODUCT_CONTEXT('part definition',#33078,'mechanical');
#33085=PRODUCT('Access Door Cover','Access Door Cover',$,(#33079));
#33098=PRESENTATION_STYLE_ASSIGNMENT((#33104));
#33104=SURFACE_STYLE_USAGE(.BOTH.,#33110);
#33110=SURFACE_SIDE_STYLE('',(#33116));
#33116=SURFACE_STYLE_FILL_AREA(#33122);
#33122=FILL_AREA_STYLE('Opaque(227,224,212)',(#33128));
#33128=FILL_AREA_STYLE_COLOUR('Opaque(227,224,212)',#33134);
#33134=COLOUR_RGB('Opaque(227,224,212)',0.890196078431372,0.87843137254902,
0.831372549019608);
ENDSEC;
END-ISO-10303-21;
